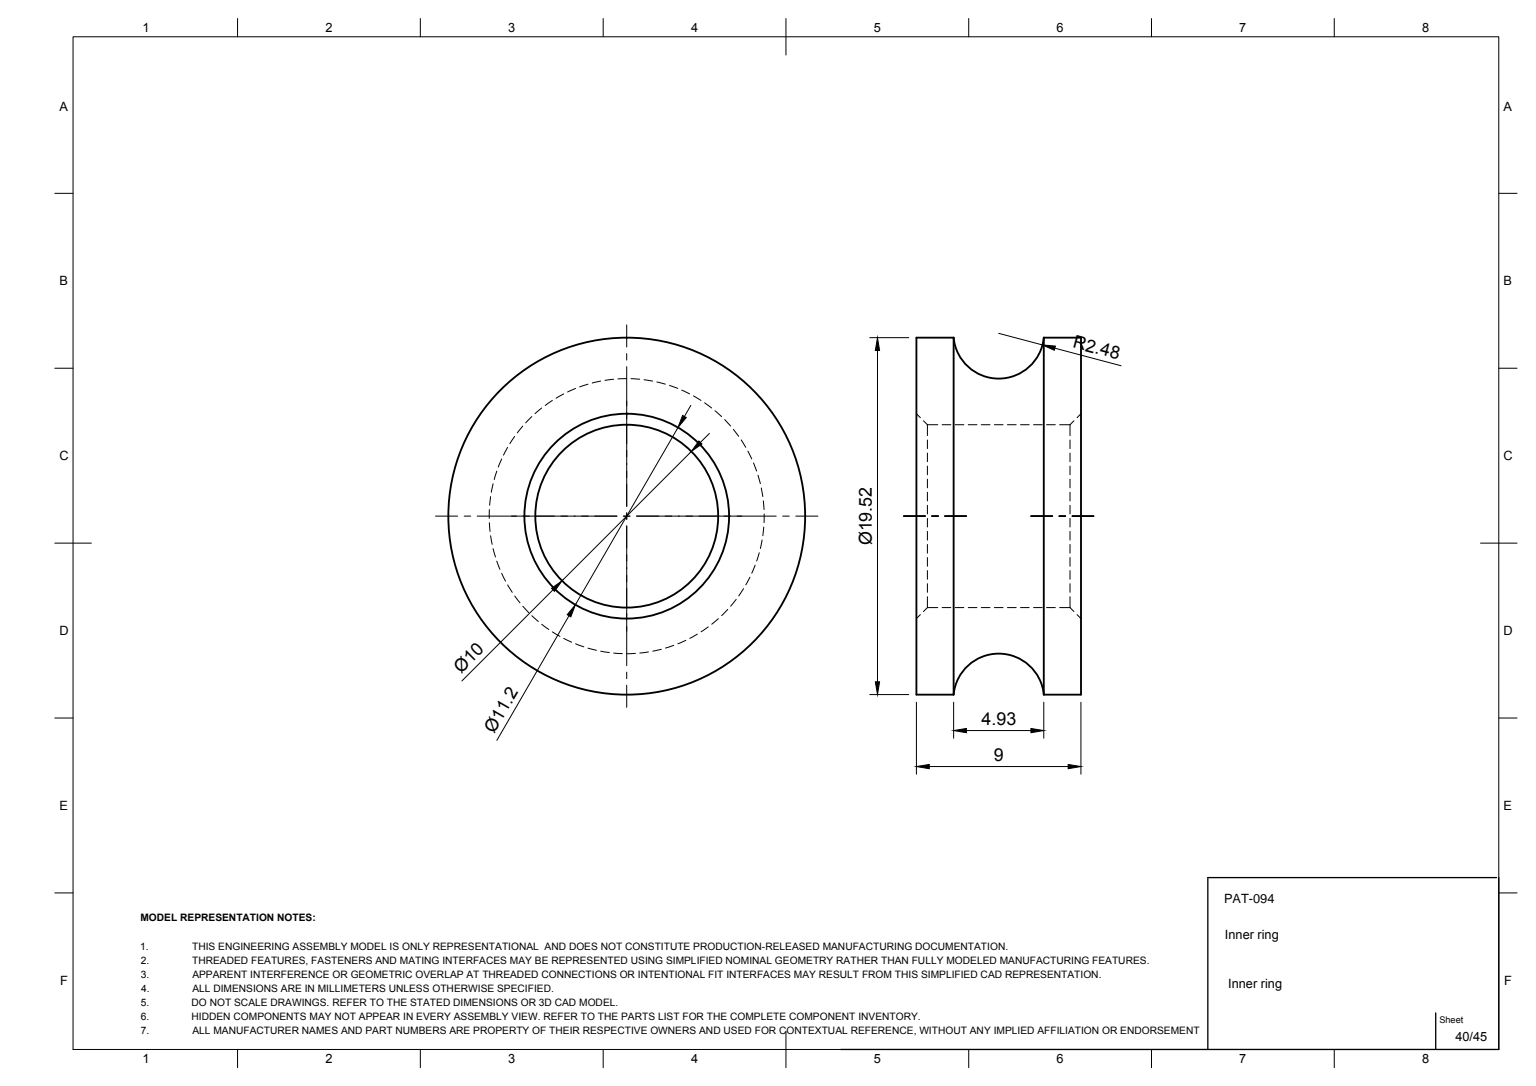
ISO-10303-21;
HEADER;
/* Generated by software containing ST-Developer
 * from STEP Tools, Inc. (www.steptools.com) 
 */

FILE_DESCRIPTION(
/* description */ ('Shaft runout checking stand'),
/* implementation_level */ '2;1');

FILE_NAME(
/* name */ 'Inner ring.step',
/* time_stamp */ '2026-11-02T21:12:33-08:00',
/* author */ (''),
/* organization */ (''),
/* preprocessor_version */ 'ST-DEVELOPER v20.2',
/* originating_system */ 'Autodesk Translation Framework v15.17.0.0',
/* authorisation */ '');

FILE_SCHEMA (('AUTOMOTIVE_DESIGN { 1 0 10303 214 3 1 1 }'));
ENDSEC;

DATA;
#10=MECHANICAL_DESIGN_GEOMETRIC_PRESENTATION_REPRESENTATION('',(#498),#11748);
#27=TOROIDAL_SURFACE('',#7323,1.,0.247676);
#371=CONICAL_SURFACE('',#7334,0.53,0.785398163397448);
#372=CONICAL_SURFACE('',#7341,0.53,0.785398163397448);
#412=SHAPE_REPRESENTATION_RELATIONSHIP('SRR','None',#11964,#455);
#455=ADVANCED_BREP_SHAPE_REPRESENTATION('',(#546),#11740);
#498=STYLED_ITEM('',(#12170),#546);
#546=MANIFOLD_SOLID_BREP('Body1',#6244);
#658=FACE_BOUND('',#1812,.T.);
#659=FACE_BOUND('',#1815,.T.);
#854=CIRCLE('',#7324,0.976185);
#855=CIRCLE('',#7325,0.976185);
#856=CIRCLE('',#7326,0.247676);
#857=CIRCLE('',#7327,0.976185);
#858=CIRCLE('',#7328,0.976185);
#859=CIRCLE('',#7330,0.976185);
#860=CIRCLE('',#7332,0.5);
#861=CIRCLE('',#7333,0.5);
#862=CIRCLE('',#7335,0.56);
#863=CIRCLE('',#7338,0.976185);
#864=CIRCLE('',#7340,0.56);
#1020=CYLINDRICAL_SURFACE('',#7329,0.976185);
#1021=CYLINDRICAL_SURFACE('',#7331,0.5);
#1022=CYLINDRICAL_SURFACE('',#7337,0.976185);
#1343=FACE_OUTER_BOUND('',#1807,.T.);
#1344=FACE_OUTER_BOUND('',#1808,.T.);
#1345=FACE_OUTER_BOUND('',#1809,.T.);
#1346=FACE_OUTER_BOUND('',#1810,.T.);
#1347=FACE_OUTER_BOUND('',#1811,.T.);
#1348=FACE_OUTER_BOUND('',#1813,.T.);
#1349=FACE_OUTER_BOUND('',#1814,.T.);
#1350=FACE_OUTER_BOUND('',#1816,.T.);
#1807=EDGE_LOOP('',(#5356,#5357,#5358,#5359,#5360,#5361));
#1808=EDGE_LOOP('',(#5362,#5363,#5364,#5365,#5366));
#1809=EDGE_LOOP('',(#5367,#5368,#5369,#5370));
#1810=EDGE_LOOP('',(#5371,#5372,#5373,#5374));
#1811=EDGE_LOOP('',(#5375));
#1812=EDGE_LOOP('',(#5376));
#1813=EDGE_LOOP('',(#5377,#5378,#5379,#5380,#5381));
#1814=EDGE_LOOP('',(#5382));
#1815=EDGE_LOOP('',(#5383));
#1816=EDGE_LOOP('',(#5384,#5385,#5386,#5387));
#2330=LINE('',#11024,#2797);
#2331=LINE('',#11030,#2798);
#2332=LINE('',#11034,#2799);
#2333=LINE('',#11040,#2800);
#2334=LINE('',#11045,#2801);
#2797=VECTOR('',#9129,0.976185);
#2798=VECTOR('',#9136,0.5);
#2799=VECTOR('',#9141,0.53);
#2800=VECTOR('',#9150,0.976185);
#2801=VECTOR('',#9157,0.53);
#3238=VERTEX_POINT('',#11013);
#3239=VERTEX_POINT('',#11014);
#3240=VERTEX_POINT('',#11017);
#3241=VERTEX_POINT('',#11019);
#3242=VERTEX_POINT('',#11023);
#3243=VERTEX_POINT('',#11027);
#3244=VERTEX_POINT('',#11029);
#3245=VERTEX_POINT('',#11033);
#3246=VERTEX_POINT('',#11038);
#3247=VERTEX_POINT('',#11042);
#3964=EDGE_CURVE('',#3238,#3239,#854,.T.);
#3965=EDGE_CURVE('',#3239,#3238,#855,.T.);
#3966=EDGE_CURVE('',#3239,#3240,#856,.T.);
#3967=EDGE_CURVE('',#3241,#3240,#857,.T.);
#3968=EDGE_CURVE('',#3240,#3241,#858,.T.);
#3969=EDGE_CURVE('',#3241,#3242,#2330,.T.);
#3970=EDGE_CURVE('',#3242,#3242,#859,.T.);
#3971=EDGE_CURVE('',#3243,#3243,#860,.T.);
#3972=EDGE_CURVE('',#3243,#3244,#2331,.T.);
#3973=EDGE_CURVE('',#3244,#3244,#861,.T.);
#3974=EDGE_CURVE('',#3244,#3245,#2332,.T.);
#3975=EDGE_CURVE('',#3245,#3245,#862,.T.);
#3976=EDGE_CURVE('',#3246,#3246,#863,.T.);
#3977=EDGE_CURVE('',#3246,#3238,#2333,.T.);
#3978=EDGE_CURVE('',#3247,#3247,#864,.T.);
#3979=EDGE_CURVE('',#3247,#3243,#2334,.T.);
#5356=ORIENTED_EDGE('',*,*,#3964,.F.);
#5357=ORIENTED_EDGE('',*,*,#3965,.F.);
#5358=ORIENTED_EDGE('',*,*,#3966,.T.);
#5359=ORIENTED_EDGE('',*,*,#3967,.F.);
#5360=ORIENTED_EDGE('',*,*,#3968,.F.);
#5361=ORIENTED_EDGE('',*,*,#3966,.F.);
#5362=ORIENTED_EDGE('',*,*,#3967,.T.);
#5363=ORIENTED_EDGE('',*,*,#3968,.T.);
#5364=ORIENTED_EDGE('',*,*,#3969,.T.);
#5365=ORIENTED_EDGE('',*,*,#3970,.T.);
#5366=ORIENTED_EDGE('',*,*,#3969,.F.);
#5367=ORIENTED_EDGE('',*,*,#3971,.T.);
#5368=ORIENTED_EDGE('',*,*,#3972,.T.);
#5369=ORIENTED_EDGE('',*,*,#3973,.F.);
#5370=ORIENTED_EDGE('',*,*,#3972,.F.);
#5371=ORIENTED_EDGE('',*,*,#3973,.T.);
#5372=ORIENTED_EDGE('',*,*,#3974,.T.);
#5373=ORIENTED_EDGE('',*,*,#3975,.F.);
#5374=ORIENTED_EDGE('',*,*,#3974,.F.);
#5375=ORIENTED_EDGE('',*,*,#3970,.F.);
#5376=ORIENTED_EDGE('',*,*,#3975,.T.);
#5377=ORIENTED_EDGE('',*,*,#3976,.F.);
#5378=ORIENTED_EDGE('',*,*,#3977,.T.);
#5379=ORIENTED_EDGE('',*,*,#3964,.T.);
#5380=ORIENTED_EDGE('',*,*,#3965,.T.);
#5381=ORIENTED_EDGE('',*,*,#3977,.F.);
#5382=ORIENTED_EDGE('',*,*,#3976,.T.);
#5383=ORIENTED_EDGE('',*,*,#3978,.F.);
#5384=ORIENTED_EDGE('',*,*,#3978,.T.);
#5385=ORIENTED_EDGE('',*,*,#3979,.T.);
#5386=ORIENTED_EDGE('',*,*,#3971,.F.);
#5387=ORIENTED_EDGE('',*,*,#3979,.F.);
#5815=PLANE('',#7336);
#5816=PLANE('',#7339);
#6143=ADVANCED_FACE('',(#1343),#27,.F.);
#6144=ADVANCED_FACE('',(#1344),#1020,.T.);
#6145=ADVANCED_FACE('',(#1345),#1021,.F.);
#6146=ADVANCED_FACE('',(#1346),#371,.F.);
#6147=ADVANCED_FACE('',(#1347,#658),#5815,.T.);
#6148=ADVANCED_FACE('',(#1348),#1022,.T.);
#6149=ADVANCED_FACE('',(#1349,#659),#5816,.T.);
#6150=ADVANCED_FACE('',(#1350),#372,.F.);
#6244=CLOSED_SHELL('',(#6143,#6144,#6145,#6146,#6147,#6148,#6149,#6150));
#7322=AXIS2_PLACEMENT_3D('',#11011,#9113,#9114);
#7323=AXIS2_PLACEMENT_3D('',#11012,#9115,#9116);
#7324=AXIS2_PLACEMENT_3D('',#11015,#9117,#9118);
#7325=AXIS2_PLACEMENT_3D('',#11016,#9119,#9120);
#7326=AXIS2_PLACEMENT_3D('',#11018,#9121,#9122);
#7327=AXIS2_PLACEMENT_3D('',#11020,#9123,#9124);
#7328=AXIS2_PLACEMENT_3D('',#11021,#9125,#9126);
#7329=AXIS2_PLACEMENT_3D('',#11022,#9127,#9128);
#7330=AXIS2_PLACEMENT_3D('',#11025,#9130,#9131);
#7331=AXIS2_PLACEMENT_3D('',#11026,#9132,#9133);
#7332=AXIS2_PLACEMENT_3D('',#11028,#9134,#9135);
#7333=AXIS2_PLACEMENT_3D('',#11031,#9137,#9138);
#7334=AXIS2_PLACEMENT_3D('',#11032,#9139,#9140);
#7335=AXIS2_PLACEMENT_3D('',#11035,#9142,#9143);
#7336=AXIS2_PLACEMENT_3D('',#11036,#9144,#9145);
#7337=AXIS2_PLACEMENT_3D('',#11037,#9146,#9147);
#7338=AXIS2_PLACEMENT_3D('',#11039,#9148,#9149);
#7339=AXIS2_PLACEMENT_3D('',#11041,#9151,#9152);
#7340=AXIS2_PLACEMENT_3D('',#11043,#9153,#9154);
#7341=AXIS2_PLACEMENT_3D('',#11044,#9155,#9156);
#9113=DIRECTION('axis',(0.,0.,1.));
#9114=DIRECTION('refdir',(1.,0.,0.));
#9115=DIRECTION('center_axis',(0.,-1.,0.));
#9116=DIRECTION('ref_axis',(0.,0.,-1.));
#9117=DIRECTION('center_axis',(0.,-1.,0.));
#9118=DIRECTION('ref_axis',(1.,0.,0.));
#9119=DIRECTION('center_axis',(0.,-1.,0.));
#9120=DIRECTION('ref_axis',(1.,0.,0.));
#9121=DIRECTION('center_axis',(1.,0.,1.22464679914735E-16));
#9122=DIRECTION('ref_axis',(-1.22464679914735E-16,0.,1.));
#9123=DIRECTION('center_axis',(0.,1.,0.));
#9124=DIRECTION('ref_axis',(1.,0.,0.));
#9125=DIRECTION('center_axis',(0.,1.,0.));
#9126=DIRECTION('ref_axis',(1.,0.,0.));
#9127=DIRECTION('center_axis',(0.,-1.,0.));
#9128=DIRECTION('ref_axis',(1.,0.,0.));
#9129=DIRECTION('',(0.,1.,0.));
#9130=DIRECTION('center_axis',(0.,-1.,0.));
#9131=DIRECTION('ref_axis',(1.,0.,0.));
#9132=DIRECTION('center_axis',(0.,-1.,0.));
#9133=DIRECTION('ref_axis',(1.,0.,0.));
#9134=DIRECTION('center_axis',(0.,-1.,0.));
#9135=DIRECTION('ref_axis',(1.,0.,0.));
#9136=DIRECTION('',(0.,1.,0.));
#9137=DIRECTION('center_axis',(0.,-1.,0.));
#9138=DIRECTION('ref_axis',(1.,0.,0.));
#9139=DIRECTION('center_axis',(0.,1.,0.));
#9140=DIRECTION('ref_axis',(1.,0.,0.));
#9141=DIRECTION('',(-0.707106781186547,0.707106781186548,-8.65956056235493E-17));
#9142=DIRECTION('center_axis',(0.,-1.,0.));
#9143=DIRECTION('ref_axis',(1.,0.,0.));
#9144=DIRECTION('center_axis',(0.,1.,0.));
#9145=DIRECTION('ref_axis',(0.,0.,1.));
#9146=DIRECTION('center_axis',(0.,-1.,0.));
#9147=DIRECTION('ref_axis',(1.,0.,0.));
#9148=DIRECTION('center_axis',(0.,-1.,0.));
#9149=DIRECTION('ref_axis',(1.,0.,0.));
#9150=DIRECTION('',(0.,1.,0.));
#9151=DIRECTION('center_axis',(0.,-1.,0.));
#9152=DIRECTION('ref_axis',(0.,0.,-1.));
#9153=DIRECTION('center_axis',(0.,-1.,0.));
#9154=DIRECTION('ref_axis',(1.,0.,0.));
#9155=DIRECTION('center_axis',(0.,-1.,0.));
#9156=DIRECTION('ref_axis',(1.,0.,0.));
#9157=DIRECTION('',(0.707106781186547,0.707106781186548,8.65956056235493E-17));
#11011=CARTESIAN_POINT('',(0.,0.,0.));
#11012=CARTESIAN_POINT('Origin',(0.,0.,0.));
#11013=CARTESIAN_POINT('',(-0.976185,-0.246528389340863,-1.19548183562566E-16));
#11014=CARTESIAN_POINT('',(-1.19548183562566E-16,-0.246528389340863,0.976185));
#11015=CARTESIAN_POINT('Origin',(0.,-0.246528389340863,0.));
#11016=CARTESIAN_POINT('Origin',(0.,-0.246528389340863,0.));
#11017=CARTESIAN_POINT('',(-1.19548183562566E-16,0.246528389340863,0.976185));
#11018=CARTESIAN_POINT('Origin',(-1.22464679914735E-16,0.,1.));
#11019=CARTESIAN_POINT('',(-0.976185,0.246528389340863,1.19548183562566E-16));
#11020=CARTESIAN_POINT('Origin',(0.,0.246528389340863,0.));
#11021=CARTESIAN_POINT('Origin',(0.,0.246528389340863,0.));
#11022=CARTESIAN_POINT('Origin',(0.,0.,0.));
#11023=CARTESIAN_POINT('',(-0.976185,0.45,-1.19548183562566E-16));
#11024=CARTESIAN_POINT('',(-0.976185,0.,-1.19548183562566E-16));
#11025=CARTESIAN_POINT('Origin',(0.,0.45,0.));
#11026=CARTESIAN_POINT('Origin',(0.,0.,0.));
#11027=CARTESIAN_POINT('',(-0.5,-0.39,-6.12323399573677E-17));
#11028=CARTESIAN_POINT('Origin',(0.,-0.39,0.));
#11029=CARTESIAN_POINT('',(-0.5,0.39,-6.12323399573677E-17));
#11030=CARTESIAN_POINT('',(-0.5,0.,-6.12323399573677E-17));
#11031=CARTESIAN_POINT('Origin',(0.,0.39,0.));
#11032=CARTESIAN_POINT('Origin',(0.,0.42,0.));
#11033=CARTESIAN_POINT('',(-0.56,0.45,-6.85802207522518E-17));
#11034=CARTESIAN_POINT('',(-0.53,0.42,-6.49062803548097E-17));
#11035=CARTESIAN_POINT('Origin',(0.,0.45,0.));
#11036=CARTESIAN_POINT('Origin',(0.976185,0.45,0.));
#11037=CARTESIAN_POINT('Origin',(0.,0.,0.));
#11038=CARTESIAN_POINT('',(-0.976185,-0.45,-1.19548183562566E-16));
#11039=CARTESIAN_POINT('Origin',(0.,-0.45,0.));
#11040=CARTESIAN_POINT('',(-0.976185,0.,-1.19548183562566E-16));
#11041=CARTESIAN_POINT('Origin',(0.56,-0.45,0.));
#11042=CARTESIAN_POINT('',(-0.56,-0.45,-6.85802207522518E-17));
#11043=CARTESIAN_POINT('Origin',(0.,-0.45,0.));
#11044=CARTESIAN_POINT('Origin',(0.,-0.42,0.));
#11045=CARTESIAN_POINT('',(-0.53,-0.42,-6.49062803548097E-17));
#11691=UNCERTAINTY_MEASURE_WITH_UNIT(LENGTH_MEASURE(0.001),#11749,
'DISTANCE_ACCURACY_VALUE',
'Maximum model space distance between geometric entities at asserted c
onnectivities');
#11699=UNCERTAINTY_MEASURE_WITH_UNIT(LENGTH_MEASURE(0.001),#11749,
'DISTANCE_ACCURACY_VALUE',
'Maximum model space distance between geometric entities at asserted c
onnectivities');
#11740=(
GEOMETRIC_REPRESENTATION_CONTEXT(3)
GLOBAL_UNCERTAINTY_ASSIGNED_CONTEXT((#11691))
GLOBAL_UNIT_ASSIGNED_CONTEXT((#11749,#11751,#11752))
REPRESENTATION_CONTEXT('','3D')
);
#11748=(
GEOMETRIC_REPRESENTATION_CONTEXT(3)
GLOBAL_UNCERTAINTY_ASSIGNED_CONTEXT((#11699))
GLOBAL_UNIT_ASSIGNED_CONTEXT((#11749,#11751,#11752))
REPRESENTATION_CONTEXT('','3D')
);
#11749=(
LENGTH_UNIT()
NAMED_UNIT(*)
SI_UNIT(.CENTI.,.METRE.)
);
#11751=(
NAMED_UNIT(*)
PLANE_ANGLE_UNIT()
SI_UNIT($,.RADIAN.)
);
#11752=(
NAMED_UNIT(*)
SI_UNIT($,.STERADIAN.)
SOLID_ANGLE_UNIT()
);
#11793=SHAPE_DEFINITION_REPRESENTATION(#11901,#11964);
#11901=PRODUCT_DEFINITION_SHAPE('',$,#12013);
#11964=SHAPE_REPRESENTATION('',(#7322),#11740);
#11972=PRODUCT_DEFINITION_CONTEXT('part definition',#12118,'design');
#12013=PRODUCT_DEFINITION('Inner ring','Inner ring',#12061,#11972);
#12061=PRODUCT_DEFINITION_FORMATION('',$,#12160);
#12118=APPLICATION_CONTEXT(
'Core Data for Automotive Mechanical Design Process');
#12119=PRODUCT_CONTEXT('part definition',#12118,'mechanical');
#12160=PRODUCT('Inner ring','Inner ring','Inner ring',(#12119));
#12170=PRESENTATION_STYLE_ASSIGNMENT((#12175));
#12175=SURFACE_STYLE_USAGE(.BOTH.,#12180);
#12180=SURFACE_SIDE_STYLE('',(#12185));
#12185=SURFACE_STYLE_FILL_AREA(#12190);
#12190=FILL_AREA_STYLE('CAD Library Painted - Steel gray',(#12195));
#12195=FILL_AREA_STYLE_COLOUR('CAD Library Painted - Steel gray',#12200);
#12200=COLOUR_RGB('CAD Library Painted - Steel gray',0.592156862745098,
0.631372549019608,0.67843137254902);
ENDSEC;
END-ISO-10303-21;
